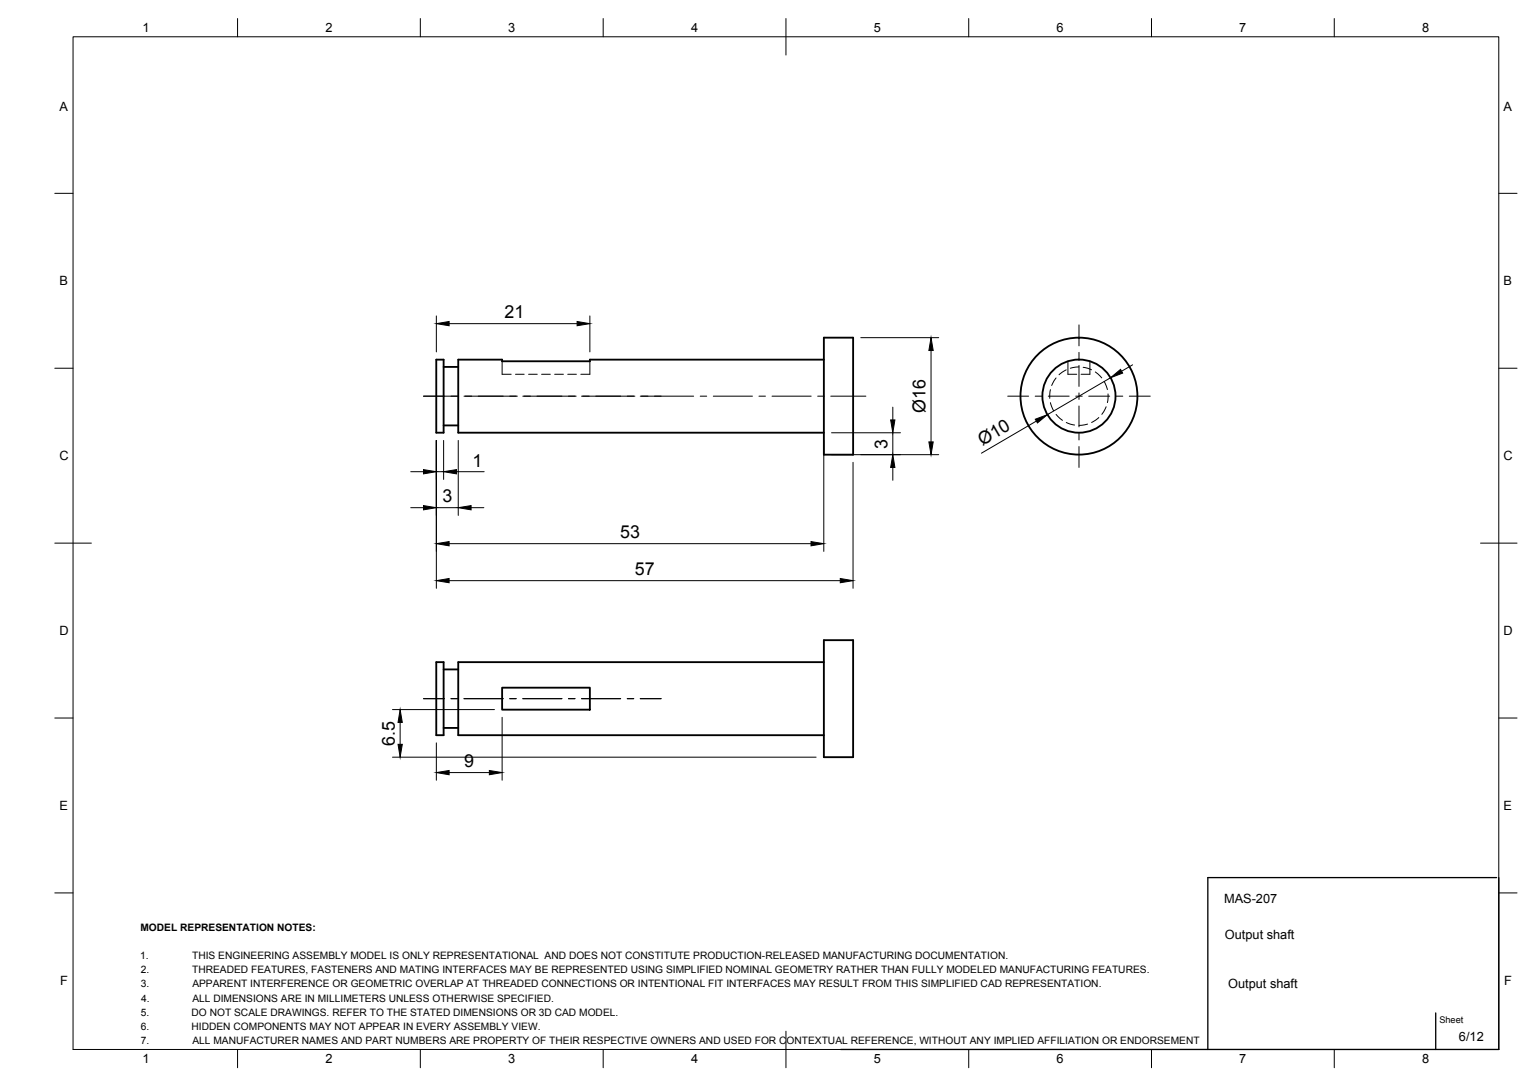
ISO-10303-21;
HEADER;
/* Generated by software containing ST-Developer
 * from STEP Tools, Inc. (www.steptools.com) 
 */

FILE_DESCRIPTION(
/* description */ ('Independent six-slot Geneva indexer. Center distance100, drive radius
50, 60degree indexing per input revolution with120degree engagement an
d240degree dwell. Native machined concave locking faces and relieved d
isk; replaceable retained drive pin; keyed output shaft. Geometry traj
ectory checks use calculated indexing positions, not a contact-dynamic
s simulation. No load or production rating assigned.'),
/* implementation_level */ '2;1');

FILE_NAME(
/* name */ 'Output shaft.step',
/* time_stamp */ '2026-11-09T17:53:22-08:00',
/* author */ (''),
/* organization */ (''),
/* preprocessor_version */ 'ST-DEVELOPER v20.2',
/* originating_system */ 'Autodesk Translation Framework v15.17.0.0',
/* authorisation */ '');

FILE_SCHEMA (('AUTOMOTIVE_DESIGN { 1 0 10303 214 3 1 1 }'));
ENDSEC;

DATA;
#10=MECHANICAL_DESIGN_GEOMETRIC_PRESENTATION_REPRESENTATION('',(#104),#4149);
#82=SHAPE_REPRESENTATION_RELATIONSHIP('SRR','None',#4199,#93);
#93=ADVANCED_BREP_SHAPE_REPRESENTATION('',(#115),#4141);
#104=STYLED_ITEM('',(#4263),#115);
#115=MANIFOLD_SOLID_BREP('Body1',#2298);
#144=FACE_BOUND('',#483,.T.);
#145=FACE_BOUND('',#485,.T.);
#146=FACE_BOUND('',#488,.T.);
#147=FACE_BOUND('',#492,.T.);
#203=PLANE('',#2596);
#204=PLANE('',#2597);
#205=PLANE('',#2599);
#206=PLANE('',#2600);
#207=PLANE('',#2601);
#208=PLANE('',#2606);
#209=PLANE('',#2608);
#210=PLANE('',#2612);
#211=PLANE('',#2617);
#212=PLANE('',#2619);
#319=FACE_OUTER_BOUND('',#476,.T.);
#320=FACE_OUTER_BOUND('',#477,.T.);
#321=FACE_OUTER_BOUND('',#478,.T.);
#322=FACE_OUTER_BOUND('',#479,.T.);
#323=FACE_OUTER_BOUND('',#480,.T.);
#324=FACE_OUTER_BOUND('',#481,.T.);
#325=FACE_OUTER_BOUND('',#482,.T.);
#326=FACE_OUTER_BOUND('',#484,.T.);
#327=FACE_OUTER_BOUND('',#486,.T.);
#328=FACE_OUTER_BOUND('',#487,.T.);
#329=FACE_OUTER_BOUND('',#489,.T.);
#330=FACE_OUTER_BOUND('',#490,.T.);
#331=FACE_OUTER_BOUND('',#491,.T.);
#332=FACE_OUTER_BOUND('',#493,.T.);
#476=EDGE_LOOP('',(#1920,#1921,#1922,#1923));
#477=EDGE_LOOP('',(#1924,#1925,#1926,#1927));
#478=EDGE_LOOP('',(#1928,#1929,#1930,#1931));
#479=EDGE_LOOP('',(#1932,#1933,#1934,#1935));
#480=EDGE_LOOP('',(#1936,#1937,#1938,#1939));
#481=EDGE_LOOP('',(#1940,#1941,#1942,#1943));
#482=EDGE_LOOP('',(#1944));
#483=EDGE_LOOP('',(#1945));
#484=EDGE_LOOP('',(#1946));
#485=EDGE_LOOP('',(#1947));
#486=EDGE_LOOP('',(#1948,#1949,#1950,#1951));
#487=EDGE_LOOP('',(#1952));
#488=EDGE_LOOP('',(#1953));
#489=EDGE_LOOP('',(#1954,#1955,#1956,#1957));
#490=EDGE_LOOP('',(#1958));
#491=EDGE_LOOP('',(#1959,#1960,#1961,#1962));
#492=EDGE_LOOP('',(#1963,#1964,#1965,#1966));
#493=EDGE_LOOP('',(#1967));
#672=LINE('',#3898,#844);
#673=LINE('',#3900,#845);
#674=LINE('',#3902,#846);
#675=LINE('',#3903,#847);
#676=LINE('',#3908,#848);
#677=LINE('',#3909,#849);
#678=LINE('',#3912,#850);
#679=LINE('',#3914,#851);
#680=LINE('',#3915,#852);
#681=LINE('',#3917,#853);
#682=LINE('',#3924,#854);
#683=LINE('',#3935,#855);
#684=LINE('',#3943,#856);
#685=LINE('',#3947,#857);
#844=VECTOR('',#3179,10.);
#845=VECTOR('',#3180,10.);
#846=VECTOR('',#3181,10.);
#847=VECTOR('',#3182,10.);
#848=VECTOR('',#3187,10.);
#849=VECTOR('',#3188,10.);
#850=VECTOR('',#3191,10.);
#851=VECTOR('',#3192,10.);
#852=VECTOR('',#3193,10.);
#853=VECTOR('',#3196,10.);
#854=VECTOR('',#3205,4.);
#855=VECTOR('',#3220,5.);
#856=VECTOR('',#3229,8.);
#857=VECTOR('',#3236,5.);
#974=CIRCLE('',#2598,5.);
#975=CIRCLE('',#2602,5.);
#976=CIRCLE('',#2604,4.);
#977=CIRCLE('',#2605,4.);
#978=CIRCLE('',#2607,5.);
#979=CIRCLE('',#2609,5.);
#980=CIRCLE('',#2611,5.);
#981=CIRCLE('',#2613,8.);
#982=CIRCLE('',#2614,5.);
#983=CIRCLE('',#2616,8.);
#1152=VERTEX_POINT('',#3896);
#1153=VERTEX_POINT('',#3897);
#1154=VERTEX_POINT('',#3899);
#1155=VERTEX_POINT('',#3901);
#1156=VERTEX_POINT('',#3905);
#1157=VERTEX_POINT('',#3907);
#1158=VERTEX_POINT('',#3911);
#1159=VERTEX_POINT('',#3913);
#1160=VERTEX_POINT('',#3921);
#1161=VERTEX_POINT('',#3923);
#1162=VERTEX_POINT('',#3927);
#1163=VERTEX_POINT('',#3930);
#1164=VERTEX_POINT('',#3933);
#1165=VERTEX_POINT('',#3937);
#1166=VERTEX_POINT('',#3939);
#1167=VERTEX_POINT('',#3942);
#1418=EDGE_CURVE('',#1152,#1153,#672,.T.);
#1419=EDGE_CURVE('',#1152,#1154,#673,.T.);
#1420=EDGE_CURVE('',#1155,#1154,#674,.T.);
#1421=EDGE_CURVE('',#1155,#1153,#675,.T.);
#1422=EDGE_CURVE('',#1153,#1156,#974,.T.);
#1423=EDGE_CURVE('',#1157,#1155,#676,.T.);
#1424=EDGE_CURVE('',#1156,#1157,#677,.T.);
#1425=EDGE_CURVE('',#1156,#1158,#678,.T.);
#1426=EDGE_CURVE('',#1157,#1159,#679,.T.);
#1427=EDGE_CURVE('',#1159,#1158,#680,.T.);
#1428=EDGE_CURVE('',#1154,#1159,#681,.T.);
#1429=EDGE_CURVE('',#1158,#1152,#975,.T.);
#1430=EDGE_CURVE('',#1160,#1160,#976,.T.);
#1431=EDGE_CURVE('',#1160,#1161,#682,.T.);
#1432=EDGE_CURVE('',#1161,#1161,#977,.T.);
#1433=EDGE_CURVE('',#1162,#1162,#978,.T.);
#1434=EDGE_CURVE('',#1163,#1163,#979,.T.);
#1435=EDGE_CURVE('',#1164,#1164,#980,.T.);
#1436=EDGE_CURVE('',#1164,#1163,#683,.T.);
#1437=EDGE_CURVE('',#1165,#1165,#981,.T.);
#1438=EDGE_CURVE('',#1166,#1166,#982,.T.);
#1439=EDGE_CURVE('',#1165,#1167,#684,.T.);
#1440=EDGE_CURVE('',#1167,#1167,#983,.T.);
#1441=EDGE_CURVE('',#1162,#1166,#685,.T.);
#1920=ORIENTED_EDGE('',*,*,#1418,.F.);
#1921=ORIENTED_EDGE('',*,*,#1419,.T.);
#1922=ORIENTED_EDGE('',*,*,#1420,.F.);
#1923=ORIENTED_EDGE('',*,*,#1421,.T.);
#1924=ORIENTED_EDGE('',*,*,#1422,.F.);
#1925=ORIENTED_EDGE('',*,*,#1421,.F.);
#1926=ORIENTED_EDGE('',*,*,#1423,.F.);
#1927=ORIENTED_EDGE('',*,*,#1424,.F.);
#1928=ORIENTED_EDGE('',*,*,#1425,.F.);
#1929=ORIENTED_EDGE('',*,*,#1424,.T.);
#1930=ORIENTED_EDGE('',*,*,#1426,.T.);
#1931=ORIENTED_EDGE('',*,*,#1427,.T.);
#1932=ORIENTED_EDGE('',*,*,#1423,.T.);
#1933=ORIENTED_EDGE('',*,*,#1420,.T.);
#1934=ORIENTED_EDGE('',*,*,#1428,.T.);
#1935=ORIENTED_EDGE('',*,*,#1426,.F.);
#1936=ORIENTED_EDGE('',*,*,#1429,.F.);
#1937=ORIENTED_EDGE('',*,*,#1427,.F.);
#1938=ORIENTED_EDGE('',*,*,#1428,.F.);
#1939=ORIENTED_EDGE('',*,*,#1419,.F.);
#1940=ORIENTED_EDGE('',*,*,#1430,.T.);
#1941=ORIENTED_EDGE('',*,*,#1431,.T.);
#1942=ORIENTED_EDGE('',*,*,#1432,.F.);
#1943=ORIENTED_EDGE('',*,*,#1431,.F.);
#1944=ORIENTED_EDGE('',*,*,#1433,.F.);
#1945=ORIENTED_EDGE('',*,*,#1430,.F.);
#1946=ORIENTED_EDGE('',*,*,#1434,.F.);
#1947=ORIENTED_EDGE('',*,*,#1432,.T.);
#1948=ORIENTED_EDGE('',*,*,#1435,.F.);
#1949=ORIENTED_EDGE('',*,*,#1436,.T.);
#1950=ORIENTED_EDGE('',*,*,#1434,.T.);
#1951=ORIENTED_EDGE('',*,*,#1436,.F.);
#1952=ORIENTED_EDGE('',*,*,#1437,.T.);
#1953=ORIENTED_EDGE('',*,*,#1438,.F.);
#1954=ORIENTED_EDGE('',*,*,#1437,.F.);
#1955=ORIENTED_EDGE('',*,*,#1439,.T.);
#1956=ORIENTED_EDGE('',*,*,#1440,.T.);
#1957=ORIENTED_EDGE('',*,*,#1439,.F.);
#1958=ORIENTED_EDGE('',*,*,#1440,.F.);
#1959=ORIENTED_EDGE('',*,*,#1433,.T.);
#1960=ORIENTED_EDGE('',*,*,#1441,.T.);
#1961=ORIENTED_EDGE('',*,*,#1438,.T.);
#1962=ORIENTED_EDGE('',*,*,#1441,.F.);
#1963=ORIENTED_EDGE('',*,*,#1425,.T.);
#1964=ORIENTED_EDGE('',*,*,#1429,.T.);
#1965=ORIENTED_EDGE('',*,*,#1418,.T.);
#1966=ORIENTED_EDGE('',*,*,#1422,.T.);
#1967=ORIENTED_EDGE('',*,*,#1435,.T.);
#2139=CYLINDRICAL_SURFACE('',#2603,4.);
#2140=CYLINDRICAL_SURFACE('',#2610,5.);
#2141=CYLINDRICAL_SURFACE('',#2615,8.);
#2142=CYLINDRICAL_SURFACE('',#2618,5.);
#2240=ADVANCED_FACE('',(#319),#203,.F.);
#2241=ADVANCED_FACE('',(#320),#204,.F.);
#2242=ADVANCED_FACE('',(#321),#205,.F.);
#2243=ADVANCED_FACE('',(#322),#206,.F.);
#2244=ADVANCED_FACE('',(#323),#207,.F.);
#2245=ADVANCED_FACE('',(#324),#2139,.T.);
#2246=ADVANCED_FACE('',(#325,#144),#208,.F.);
#2247=ADVANCED_FACE('',(#326,#145),#209,.F.);
#2248=ADVANCED_FACE('',(#327),#2140,.T.);
#2249=ADVANCED_FACE('',(#328,#146),#210,.T.);
#2250=ADVANCED_FACE('',(#329),#2141,.T.);
#2251=ADVANCED_FACE('',(#330),#211,.F.);
#2252=ADVANCED_FACE('',(#331,#147),#2142,.T.);
#2253=ADVANCED_FACE('',(#332),#212,.T.);
#2298=CLOSED_SHELL('',(#2240,#2241,#2242,#2243,#2244,#2245,#2246,#2247,
#2248,#2249,#2250,#2251,#2252,#2253));
#2595=AXIS2_PLACEMENT_3D('',#3894,#3175,#3176);
#2596=AXIS2_PLACEMENT_3D('',#3895,#3177,#3178);
#2597=AXIS2_PLACEMENT_3D('',#3904,#3183,#3184);
#2598=AXIS2_PLACEMENT_3D('',#3906,#3185,#3186);
#2599=AXIS2_PLACEMENT_3D('',#3910,#3189,#3190);
#2600=AXIS2_PLACEMENT_3D('',#3916,#3194,#3195);
#2601=AXIS2_PLACEMENT_3D('',#3918,#3197,#3198);
#2602=AXIS2_PLACEMENT_3D('',#3919,#3199,#3200);
#2603=AXIS2_PLACEMENT_3D('',#3920,#3201,#3202);
#2604=AXIS2_PLACEMENT_3D('',#3922,#3203,#3204);
#2605=AXIS2_PLACEMENT_3D('',#3925,#3206,#3207);
#2606=AXIS2_PLACEMENT_3D('',#3926,#3208,#3209);
#2607=AXIS2_PLACEMENT_3D('',#3928,#3210,#3211);
#2608=AXIS2_PLACEMENT_3D('',#3929,#3212,#3213);
#2609=AXIS2_PLACEMENT_3D('',#3931,#3214,#3215);
#2610=AXIS2_PLACEMENT_3D('',#3932,#3216,#3217);
#2611=AXIS2_PLACEMENT_3D('',#3934,#3218,#3219);
#2612=AXIS2_PLACEMENT_3D('',#3936,#3221,#3222);
#2613=AXIS2_PLACEMENT_3D('',#3938,#3223,#3224);
#2614=AXIS2_PLACEMENT_3D('',#3940,#3225,#3226);
#2615=AXIS2_PLACEMENT_3D('',#3941,#3227,#3228);
#2616=AXIS2_PLACEMENT_3D('',#3944,#3230,#3231);
#2617=AXIS2_PLACEMENT_3D('',#3945,#3232,#3233);
#2618=AXIS2_PLACEMENT_3D('',#3946,#3234,#3235);
#2619=AXIS2_PLACEMENT_3D('',#3948,#3237,#3238);
#3175=DIRECTION('axis',(0.,0.,1.));
#3176=DIRECTION('refdir',(1.,0.,0.));
#3177=DIRECTION('center_axis',(0.,-1.,0.));
#3178=DIRECTION('ref_axis',(-1.,0.,0.));
#3179=DIRECTION('',(0.,0.,1.));
#3180=DIRECTION('',(-1.,0.,0.));
#3181=DIRECTION('',(0.,0.,-1.));
#3182=DIRECTION('',(1.,0.,0.));
#3183=DIRECTION('center_axis',(0.,0.,1.));
#3184=DIRECTION('ref_axis',(1.,0.,0.));
#3185=DIRECTION('center_axis',(0.,0.,1.));
#3186=DIRECTION('ref_axis',(1.,0.,0.));
#3187=DIRECTION('',(0.,-1.,0.));
#3188=DIRECTION('',(-1.,0.,0.));
#3189=DIRECTION('center_axis',(0.,1.,0.));
#3190=DIRECTION('ref_axis',(1.,0.,0.));
#3191=DIRECTION('',(0.,0.,-1.));
#3192=DIRECTION('',(0.,0.,-1.));
#3193=DIRECTION('',(1.,0.,0.));
#3194=DIRECTION('center_axis',(-1.,0.,0.));
#3195=DIRECTION('ref_axis',(0.,1.,0.));
#3196=DIRECTION('',(0.,1.,0.));
#3197=DIRECTION('center_axis',(0.,0.,-1.));
#3198=DIRECTION('ref_axis',(-1.,0.,0.));
#3199=DIRECTION('center_axis',(0.,0.,-1.));
#3200=DIRECTION('ref_axis',(1.,0.,0.));
#3201=DIRECTION('center_axis',(0.,0.,1.));
#3202=DIRECTION('ref_axis',(1.,0.,0.));
#3203=DIRECTION('center_axis',(0.,0.,1.));
#3204=DIRECTION('ref_axis',(1.,0.,0.));
#3205=DIRECTION('',(0.,0.,1.));
#3206=DIRECTION('center_axis',(0.,0.,1.));
#3207=DIRECTION('ref_axis',(1.,0.,0.));
#3208=DIRECTION('center_axis',(0.,0.,-1.));
#3209=DIRECTION('ref_axis',(-1.,0.,0.));
#3210=DIRECTION('center_axis',(0.,0.,-1.));
#3211=DIRECTION('ref_axis',(1.,0.,0.));
#3212=DIRECTION('center_axis',(0.,0.,1.));
#3213=DIRECTION('ref_axis',(1.,0.,0.));
#3214=DIRECTION('center_axis',(0.,0.,1.));
#3215=DIRECTION('ref_axis',(1.,0.,0.));
#3216=DIRECTION('center_axis',(0.,0.,1.));
#3217=DIRECTION('ref_axis',(1.,0.,0.));
#3218=DIRECTION('center_axis',(0.,0.,1.));
#3219=DIRECTION('ref_axis',(1.,0.,0.));
#3220=DIRECTION('',(0.,0.,-1.));
#3221=DIRECTION('center_axis',(0.,0.,1.));
#3222=DIRECTION('ref_axis',(1.,0.,0.));
#3223=DIRECTION('center_axis',(0.,0.,1.));
#3224=DIRECTION('ref_axis',(1.,0.,0.));
#3225=DIRECTION('center_axis',(0.,0.,1.));
#3226=DIRECTION('ref_axis',(1.,0.,0.));
#3227=DIRECTION('center_axis',(0.,0.,1.));
#3228=DIRECTION('ref_axis',(1.,0.,0.));
#3229=DIRECTION('',(0.,0.,-1.));
#3230=DIRECTION('center_axis',(0.,0.,1.));
#3231=DIRECTION('ref_axis',(1.,0.,0.));
#3232=DIRECTION('center_axis',(0.,0.,1.));
#3233=DIRECTION('ref_axis',(1.,0.,0.));
#3234=DIRECTION('center_axis',(0.,0.,1.));
#3235=DIRECTION('ref_axis',(1.,0.,0.));
#3236=DIRECTION('',(0.,0.,-1.));
#3237=DIRECTION('center_axis',(0.,0.,1.));
#3238=DIRECTION('ref_axis',(1.,0.,0.));
#3894=CARTESIAN_POINT('',(0.,0.,0.));
#3895=CARTESIAN_POINT('Origin',(8.,-1.5,44.));
#3896=CARTESIAN_POINT('',(4.76969600708473,-1.5,32.));
#3897=CARTESIAN_POINT('',(4.76969600708473,-1.5,44.));
#3898=CARTESIAN_POINT('',(4.76969600708473,-1.5,0.));
#3899=CARTESIAN_POINT('',(3.,-1.5,32.));
#3900=CARTESIAN_POINT('',(3.,-1.5,32.));
#3901=CARTESIAN_POINT('',(3.,-1.5,44.));
#3902=CARTESIAN_POINT('',(3.,-1.5,44.));
#3903=CARTESIAN_POINT('',(3.,-1.5,44.));
#3904=CARTESIAN_POINT('Origin',(5.5,0.,44.));
#3905=CARTESIAN_POINT('',(4.76969600708473,1.5,44.));
#3906=CARTESIAN_POINT('Origin',(0.,0.,44.));
#3907=CARTESIAN_POINT('',(3.,1.5,44.));
#3908=CARTESIAN_POINT('',(3.,1.5,44.));
#3909=CARTESIAN_POINT('',(8.,1.5,44.));
#3910=CARTESIAN_POINT('Origin',(3.,1.5,44.));
#3911=CARTESIAN_POINT('',(4.76969600708473,1.5,32.));
#3912=CARTESIAN_POINT('',(4.76969600708473,1.5,0.));
#3913=CARTESIAN_POINT('',(3.,1.5,32.));
#3914=CARTESIAN_POINT('',(3.,1.5,44.));
#3915=CARTESIAN_POINT('',(8.,1.5,32.));
#3916=CARTESIAN_POINT('Origin',(3.,-1.5,44.));
#3917=CARTESIAN_POINT('',(3.,1.5,32.));
#3918=CARTESIAN_POINT('Origin',(5.5,0.,32.));
#3919=CARTESIAN_POINT('Origin',(0.,0.,32.));
#3920=CARTESIAN_POINT('Origin',(0.,0.,51.));
#3921=CARTESIAN_POINT('',(-4.,-4.89858719658941E-16,50.));
#3922=CARTESIAN_POINT('Origin',(0.,0.,50.));
#3923=CARTESIAN_POINT('',(-4.,-4.89858719658941E-16,52.));
#3924=CARTESIAN_POINT('',(-4.,-4.89858719658941E-16,51.));
#3925=CARTESIAN_POINT('Origin',(0.,0.,52.));
#3926=CARTESIAN_POINT('Origin',(8.,0.,50.));
#3927=CARTESIAN_POINT('',(-5.,6.12323399573677E-16,50.));
#3928=CARTESIAN_POINT('Origin',(0.,0.,50.));
#3929=CARTESIAN_POINT('Origin',(4.,0.,52.));
#3930=CARTESIAN_POINT('',(-5.,-6.12323399573677E-16,52.));
#3931=CARTESIAN_POINT('Origin',(0.,0.,52.));
#3932=CARTESIAN_POINT('Origin',(0.,0.,0.));
#3933=CARTESIAN_POINT('',(-5.,-6.12323399573677E-16,53.));
#3934=CARTESIAN_POINT('Origin',(0.,0.,53.));
#3935=CARTESIAN_POINT('',(-5.,-6.12323399573677E-16,0.));
#3936=CARTESIAN_POINT('Origin',(0.,0.,0.));
#3937=CARTESIAN_POINT('',(-8.,-9.79717439317883E-16,0.));
#3938=CARTESIAN_POINT('Origin',(0.,0.,0.));
#3939=CARTESIAN_POINT('',(-5.,-6.12323399573677E-16,0.));
#3940=CARTESIAN_POINT('Origin',(0.,0.,0.));
#3941=CARTESIAN_POINT('Origin',(0.,0.,-4.));
#3942=CARTESIAN_POINT('',(-8.,-9.79717439317883E-16,-4.));
#3943=CARTESIAN_POINT('',(-8.,-9.79717439317883E-16,-4.));
#3944=CARTESIAN_POINT('Origin',(0.,0.,-4.));
#3945=CARTESIAN_POINT('Origin',(0.,0.,-4.));
#3946=CARTESIAN_POINT('Origin',(0.,0.,0.));
#3947=CARTESIAN_POINT('',(-5.,-6.12323399573677E-16,0.));
#3948=CARTESIAN_POINT('Origin',(0.,0.,53.));
#4128=UNCERTAINTY_MEASURE_WITH_UNIT(LENGTH_MEASURE(0.01),#4150,
'DISTANCE_ACCURACY_VALUE',
'Maximum model space distance between geometric entities at asserted c
onnectivities');
#4136=UNCERTAINTY_MEASURE_WITH_UNIT(LENGTH_MEASURE(0.01),#4150,
'DISTANCE_ACCURACY_VALUE',
'Maximum model space distance between geometric entities at asserted c
onnectivities');
#4141=(
GEOMETRIC_REPRESENTATION_CONTEXT(3)
GLOBAL_UNCERTAINTY_ASSIGNED_CONTEXT((#4128))
GLOBAL_UNIT_ASSIGNED_CONTEXT((#4150,#4152,#4153))
REPRESENTATION_CONTEXT('','3D')
);
#4149=(
GEOMETRIC_REPRESENTATION_CONTEXT(3)
GLOBAL_UNCERTAINTY_ASSIGNED_CONTEXT((#4136))
GLOBAL_UNIT_ASSIGNED_CONTEXT((#4150,#4152,#4153))
REPRESENTATION_CONTEXT('','3D')
);
#4150=(
LENGTH_UNIT()
NAMED_UNIT(*)
SI_UNIT(.MILLI.,.METRE.)
);
#4152=(
NAMED_UNIT(*)
PLANE_ANGLE_UNIT()
SI_UNIT($,.RADIAN.)
);
#4153=(
NAMED_UNIT(*)
SI_UNIT($,.STERADIAN.)
SOLID_ANGLE_UNIT()
);
#4158=SHAPE_DEFINITION_REPRESENTATION(#4170,#4199);
#4170=PRODUCT_DEFINITION_SHAPE('',$,#4212);
#4199=SHAPE_REPRESENTATION('',(#2595),#4141);
#4207=PRODUCT_DEFINITION_CONTEXT('part definition',#4245,'design');
#4212=PRODUCT_DEFINITION('Output shaft','Output shaft',#4224,#4207);
#4224=PRODUCT_DEFINITION_FORMATION('',$,#4251);
#4245=APPLICATION_CONTEXT(
'Core Data for Automotive Mechanical Design Process');
#4246=PRODUCT_CONTEXT('part definition',#4245,'mechanical');
#4251=PRODUCT('Output shaft','Output shaft','Output shaft',(#4246));
#4263=PRESENTATION_STYLE_ASSIGNMENT((#4273));
#4273=SURFACE_STYLE_USAGE(.BOTH.,#4283);
#4283=SURFACE_SIDE_STYLE('',(#4293));
#4293=SURFACE_STYLE_FILL_AREA(#4303);
#4303=FILL_AREA_STYLE('Pivot gray',(#4313));
#4313=FILL_AREA_STYLE_COLOUR('Pivot gray',#4323);
#4323=COLOUR_RGB('Pivot gray',0.407843137254902,0.447058823529412,0.498039215686275);
ENDSEC;
END-ISO-10303-21;
